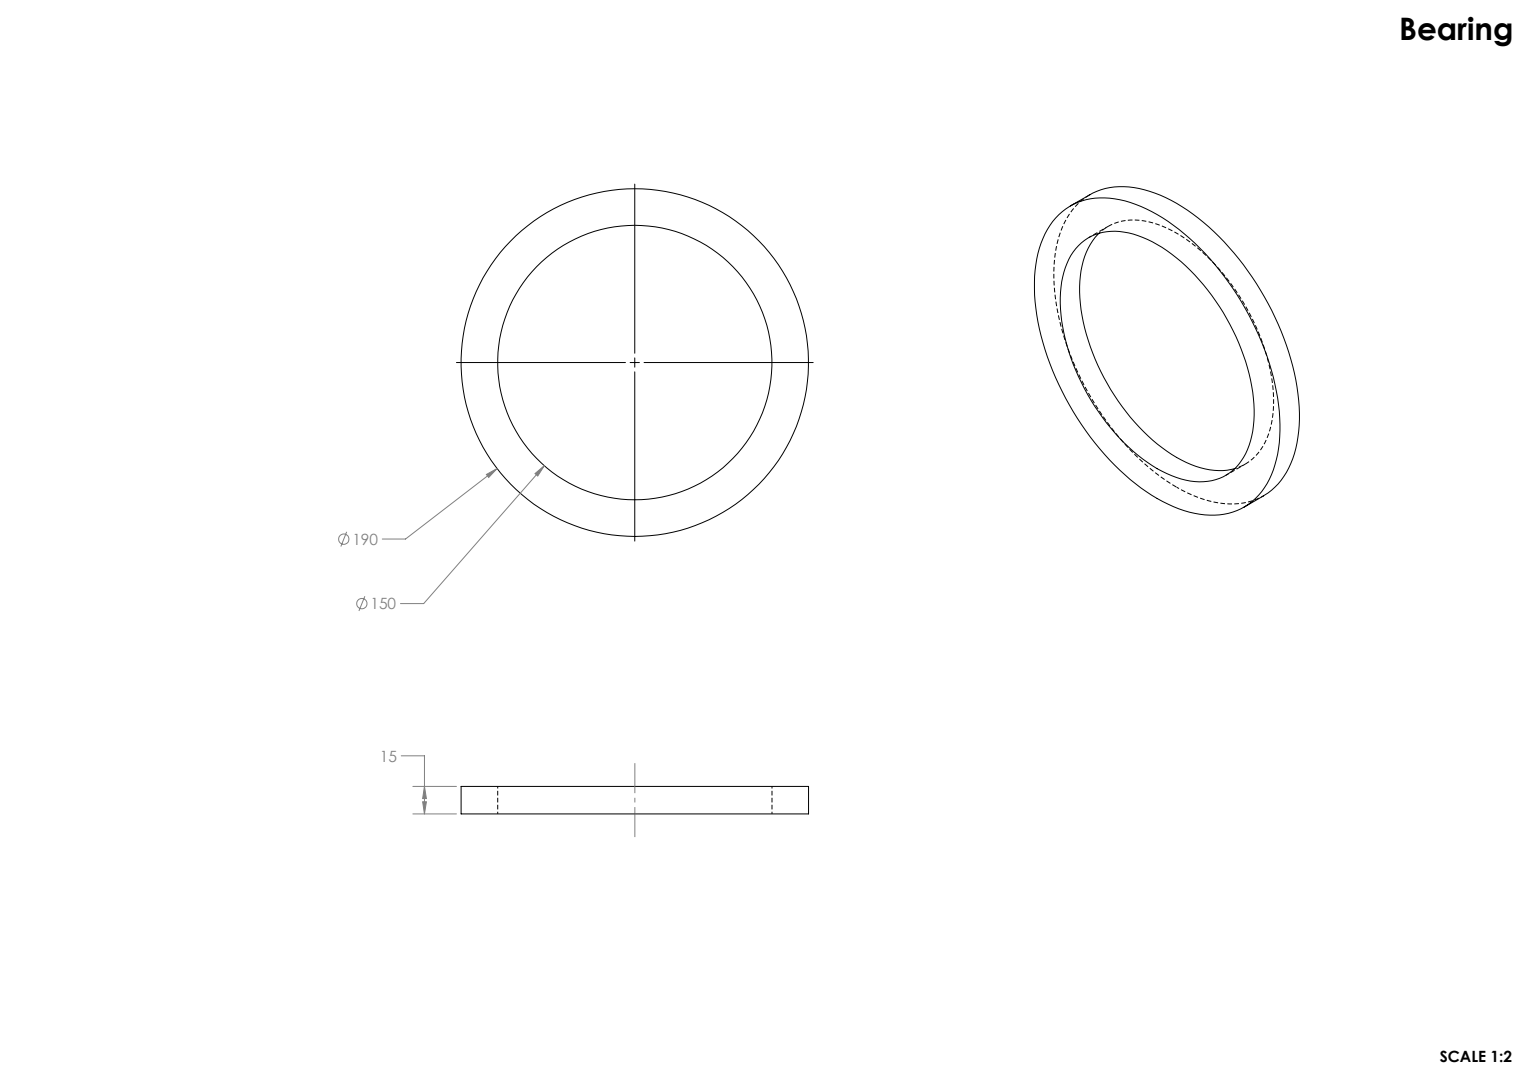
ISO-10303-21;
HEADER;
FILE_DESCRIPTION (('STEP AP214'),
    '1' );
FILE_NAME ('Bearing.step',
    '2026-10-28T15:55:38',
    ( '' ),
    ( '' ),
    'SwSTEP 2.0',
    'SolidWorks 2025',
    '' );
FILE_SCHEMA (( 'AUTOMOTIVE_DESIGN' ));
ENDSEC;

DATA;
#36=CYLINDRICAL_SURFACE ( 'NONE', #7648, 95.00000000000001421 ) ;
#43=DIRECTION ( 'NONE',  ( 0.000000000000000000, 0.000000000000000000, 1.000000000000000000 ) ) ;
#170=DIRECTION ( 'NONE',  ( 1.000000000000000000, 0.000000000000000000, 0.000000000000000000 ) ) ;
#319=CIRCLE ( 'NONE', #6386, 95.00000000000001421 ) ;
#459=DIRECTION ( 'NONE',  ( 1.000000000000000000, 0.000000000000000000, 0.000000000000000000 ) ) ;
#466=EDGE_LOOP ( 'NONE', ( #8090, #6345 ) ) ;
#470=EDGE_CURVE ( 'NONE', #8314, #877, #319, .T. ) ;
#507=AXIS2_PLACEMENT_3D ( 'NONE', #6558, #3976, #170 ) ;
#604=DIRECTION ( 'NONE',  ( -1.000000000000000000, 0.000000000000000000, 0.000000000000000000 ) ) ;
#729=CLOSED_SHELL ( 'NONE', ( #3816, #7770, #7786, #6914, #1126, #1756 ) ) ;
#772=AXIS2_PLACEMENT_3D ( 'NONE', #5605, #2410, #3654 ) ;
#778=ORIENTED_EDGE ( 'NONE', *, *, #5207, .F. ) ;
#813=PRODUCT_DEFINITION_SHAPE ( 'NONE', 'NONE',  #2910 ) ;
#833=ORIENTED_EDGE ( 'NONE', *, *, #6845, .F. ) ;
#877=VERTEX_POINT ( 'NONE', #3456 ) ;
#878=DIRECTION ( 'NONE',  ( 1.000000000000000000, 0.000000000000000000, -0.000000000000000000 ) ) ;
#883=ORIENTED_EDGE ( 'NONE', *, *, #2186, .T. ) ;
#931=MANIFOLD_SOLID_BREP ( 'Boss-Extrude1', #729 ) ;
#938=CIRCLE ( 'NONE', #2552, 75.00000000000001421 ) ;
#958=( NAMED_UNIT ( * ) PLANE_ANGLE_UNIT ( ) SI_UNIT ( $, .RADIAN. ) );
#968=AXIS2_PLACEMENT_3D ( 'NONE', #5784, #1269, #459 ) ;
#994=ORIENTED_EDGE ( 'NONE', *, *, #2184, .F. ) ;
#1126=ADVANCED_FACE ( 'NONE', ( #2059 ), #36, .T. ) ;
#1133=LINE ( 'NONE', #1260, #1871 ) ;
#1160=CYLINDRICAL_SURFACE ( 'NONE', #1942, 75.00000000000001421 ) ;
#1260=CARTESIAN_POINT ( 'NONE',  ( -75.00000000000001421, 0.000000000000000000, 15.00000000000000000 ) ) ;
#1269=DIRECTION ( 'NONE',  ( 0.000000000000000000, 0.000000000000000000, 1.000000000000000000 ) ) ;
#1270=CARTESIAN_POINT ( 'NONE',  ( -75.00000000000001421, 0.000000000000000000, 0.000000000000000000 ) ) ;
#1299=AXIS2_PLACEMENT_3D ( 'NONE', #5884, #1507, #5927 ) ;
#1321=FACE_OUTER_BOUND ( 'NONE', #2841, .T. ) ;
#1388=CARTESIAN_POINT ( 'NONE',  ( 0.000000000000000000, 0.000000000000000000, 0.000000000000000000 ) ) ;
#1448=EDGE_CURVE ( 'NONE', #5626, #4012, #7736, .T. ) ;
#1507=DIRECTION ( 'NONE',  ( 0.000000000000000000, 0.000000000000000000, 1.000000000000000000 ) ) ;
#1508=( LENGTH_UNIT ( ) NAMED_UNIT ( * ) SI_UNIT ( .MILLI., .METRE. ) );
#1514=FACE_OUTER_BOUND ( 'NONE', #2180, .T. ) ;
#1549=DIRECTION ( 'NONE',  ( 0.000000000000000000, 0.000000000000000000, 1.000000000000000000 ) ) ;
#1576=ORIENTED_EDGE ( 'NONE', *, *, #470, .T. ) ;
#1718=CARTESIAN_POINT ( 'NONE',  ( -95.00000000000001421, 0.000000000000000000, 15.00000000000000000 ) ) ;
#1719=DIRECTION ( 'NONE',  ( -0.000000000000000000, -0.000000000000000000, -1.000000000000000000 ) ) ;
#1756=ADVANCED_FACE ( 'NONE', ( #1321 ), #1160, .F. ) ;
#1871=VECTOR ( 'NONE', #1719, 1000.000000000000000 ) ;
#1901=ORIENTED_EDGE ( 'NONE', *, *, #6845, .T. ) ;
#1931=PLANE ( 'NONE',  #7835 ) ;
#1942=AXIS2_PLACEMENT_3D ( 'NONE', #4989, #5072, #604 ) ;
#1999=LINE ( 'NONE', #4491, #3203 ) ;
#2059=FACE_OUTER_BOUND ( 'NONE', #4783, .T. ) ;
#2128=ORIENTED_EDGE ( 'NONE', *, *, #5048, .F. ) ;
#2180=EDGE_LOOP ( 'NONE', ( #2394, #6230 ) ) ;
#2184=EDGE_CURVE ( 'NONE', #5018, #7120, #6621, .T. ) ;
#2186=EDGE_CURVE ( 'NONE', #4012, #5626, #5543, .T. ) ;
#2227=ADVANCED_BREP_SHAPE_REPRESENTATION ( '', ( #931, #1299 ), #5023 ) ;
#2394=ORIENTED_EDGE ( 'NONE', *, *, #4348, .F. ) ;
#2410=DIRECTION ( 'NONE',  ( -0.000000000000000000, -0.000000000000000000, -1.000000000000000000 ) ) ;
#2508=DIRECTION ( 'NONE',  ( -0.000000000000000000, -0.000000000000000000, -1.000000000000000000 ) ) ;
#2552=AXIS2_PLACEMENT_3D ( 'NONE', #7127, #4450, #7042 ) ;
#2554=DIRECTION ( 'NONE',  ( -1.000000000000000000, 0.000000000000000000, 0.000000000000000000 ) ) ;
#2597=EDGE_CURVE ( 'NONE', #5626, #5018, #1133, .T. ) ;
#2762=PLANE ( 'NONE',  #6990 ) ;
#2841=EDGE_LOOP ( 'NONE', ( #3155, #883, #6890, #833 ) ) ;
#2877=CARTESIAN_POINT ( 'NONE',  ( 0.000000000000000000, 0.000000000000000000, 15.00000000000000000 ) ) ;
#2910=PRODUCT_DEFINITION ( 'UNKNOWN', '', #4750, #4112 ) ;
#2967=AXIS2_PLACEMENT_3D ( 'NONE', #4370, #3835, #6926 ) ;
#3010=CARTESIAN_POINT ( 'NONE',  ( 75.00000000000001421, 9.184850993605150311E-15, 0.000000000000000000 ) ) ;
#3045=EDGE_CURVE ( 'NONE', #4012, #7120, #1999, .T. ) ;
#3070=SHAPE_DEFINITION_REPRESENTATION ( #813, #8061 ) ;
#3119=DIRECTION ( 'NONE',  ( 1.000000000000000000, 0.000000000000000000, 0.000000000000000000 ) ) ;
#3155=ORIENTED_EDGE ( 'NONE', *, *, #3045, .F. ) ;
#3167=CARTESIAN_POINT ( 'NONE',  ( 0.000000000000000000, 0.000000000000000000, 15.00000000000000000 ) ) ;
#3203=VECTOR ( 'NONE', #4288, 1000.000000000000000 ) ;
#3250=VERTEX_POINT ( 'NONE', #1718 ) ;
#3275=LINE ( 'NONE', #6536, #3329 ) ;
#3283=ORIENTED_EDGE ( 'NONE', *, *, #2184, .T. ) ;
#3329=VECTOR ( 'NONE', #4636, 1000.000000000000000 ) ;
#3350=VERTEX_POINT ( 'NONE', #6818 ) ;
#3360=APPLICATION_CONTEXT ( 'automotive_design' ) ;
#3380=AXIS2_PLACEMENT_3D ( 'NONE', #2877, #1549, #6614 ) ;
#3432=EDGE_LOOP ( 'NONE', ( #2128, #7481, #1576, #778 ) ) ;
#3456=CARTESIAN_POINT ( 'NONE',  ( -95.00000000000001421, 0.000000000000000000, 0.000000000000000000 ) ) ;
#3499=( NAMED_UNIT ( * ) SI_UNIT ( $, .STERADIAN. ) SOLID_ANGLE_UNIT ( ) );
#3584=CIRCLE ( 'NONE', #507, 95.00000000000001421 ) ;
#3654=DIRECTION ( 'NONE',  ( -1.000000000000000000, 0.000000000000000000, 0.000000000000000000 ) ) ;
#3709=ORIENTED_EDGE ( 'NONE', *, *, #5048, .T. ) ;
#3774=FACE_OUTER_BOUND ( 'NONE', #3432, .T. ) ;
#3816=ADVANCED_FACE ( 'NONE', ( #4362 ), #4965, .F. ) ;
#3835=DIRECTION ( 'NONE',  ( 0.000000000000000000, 0.000000000000000000, 1.000000000000000000 ) ) ;
#3976=DIRECTION ( 'NONE',  ( 0.000000000000000000, 0.000000000000000000, 1.000000000000000000 ) ) ;
#4012=VERTEX_POINT ( 'NONE', #5035 ) ;
#4090=MECHANICAL_DESIGN_GEOMETRIC_PRESENTATION_REPRESENTATION('',(#5733),#8020);
#4112=PRODUCT_DEFINITION_CONTEXT ( 'detailed design', #7435, 'design' ) ;
#4134=LINE ( 'NONE', #5418, #5387 ) ;
#4288=DIRECTION ( 'NONE',  ( -0.000000000000000000, -0.000000000000000000, -1.000000000000000000 ) ) ;
#4348=EDGE_CURVE ( 'NONE', #877, #8314, #3584, .T. ) ;
#4362=FACE_OUTER_BOUND ( 'NONE', #4998, .T. ) ;
#4370=CARTESIAN_POINT ( 'NONE',  ( 0.000000000000000000, 0.000000000000000000, 15.00000000000000000 ) ) ;
#4374=CARTESIAN_POINT ( 'NONE',  ( 0.000000000000000000, 0.000000000000000000, 15.00000000000000000 ) ) ;
#4429=CYLINDRICAL_SURFACE ( 'NONE', #5257, 95.00000000000001421 ) ;
#4439=DIRECTION ( 'NONE',  ( 0.000000000000000000, 0.000000000000000000, 1.000000000000000000 ) ) ;
#4450=DIRECTION ( 'NONE',  ( 0.000000000000000000, 0.000000000000000000, 1.000000000000000000 ) ) ;
#4491=CARTESIAN_POINT ( 'NONE',  ( 75.00000000000001421, 9.184850993605150311E-15, 15.00000000000000000 ) ) ;
#4503=CARTESIAN_POINT ( 'NONE',  ( 0.000000000000000000, 0.000000000000000000, 15.00000000000000000 ) ) ;
#4636=DIRECTION ( 'NONE',  ( -0.000000000000000000, -0.000000000000000000, -1.000000000000000000 ) ) ;
#4647=DIRECTION ( 'NONE',  ( 1.000000000000000000, 0.000000000000000000, -0.000000000000000000 ) ) ;
#4750=PRODUCT_DEFINITION_FORMATION_WITH_SPECIFIED_SOURCE ( 'ANY', '', #6807, .NOT_KNOWN. ) ;
#4783=EDGE_LOOP ( 'NONE', ( #7649, #6161, #7566, #5649 ) ) ;
#4810=EDGE_LOOP ( 'NONE', ( #3283, #1901 ) ) ;
#4821=( NAMED_UNIT ( * ) PLANE_ANGLE_UNIT ( ) SI_UNIT ( $, .RADIAN. ) );
#4921=PRODUCT_CONTEXT ( 'NONE', #3360, 'mechanical' ) ;
#4965=CYLINDRICAL_SURFACE ( 'NONE', #772, 75.00000000000001421 ) ;
#4989=CARTESIAN_POINT ( 'NONE',  ( 0.000000000000000000, 0.000000000000000000, 15.00000000000000000 ) ) ;
#4998=EDGE_LOOP ( 'NONE', ( #5801, #6492, #994, #6907 ) ) ;
#5018=VERTEX_POINT ( 'NONE', #1270 ) ;
#5023=( GEOMETRIC_REPRESENTATION_CONTEXT ( 3 ) GLOBAL_UNCERTAINTY_ASSIGNED_CONTEXT ( ( #6995 ) ) GLOBAL_UNIT_ASSIGNED_CONTEXT ( ( #5461, #958, #3499 ) ) REPRESENTATION_CONTEXT ( 'NONE', 'WORKASPACE' ) );
#5035=CARTESIAN_POINT ( 'NONE',  ( 75.00000000000001421, 9.184850993605150311E-15, 15.00000000000000000 ) ) ;
#5048=EDGE_CURVE ( 'NONE', #3350, #3250, #5095, .T. ) ;
#5072=DIRECTION ( 'NONE',  ( -0.000000000000000000, -0.000000000000000000, -1.000000000000000000 ) ) ;
#5095=CIRCLE ( 'NONE', #5369, 95.00000000000001421 ) ;
#5117=FACE_OUTER_BOUND ( 'NONE', #7436, .T. ) ;
#5207=EDGE_CURVE ( 'NONE', #3250, #877, #3275, .T. ) ;
#5257=AXIS2_PLACEMENT_3D ( 'NONE', #3167, #5754, #2554 ) ;
#5369=AXIS2_PLACEMENT_3D ( 'NONE', #4374, #7699, #3119 ) ;
#5387=VECTOR ( 'NONE', #7995, 1000.000000000000000 ) ;
#5408=DIRECTION ( 'NONE',  ( 1.000000000000000000, 0.000000000000000000, 0.000000000000000000 ) ) ;
#5418=CARTESIAN_POINT ( 'NONE',  ( 95.00000000000001421, 1.163414459189985801E-14, 15.00000000000000000 ) ) ;
#5461=( LENGTH_UNIT ( ) NAMED_UNIT ( * ) SI_UNIT ( .MILLI., .METRE. ) );
#5543=CIRCLE ( 'NONE', #2967, 75.00000000000001421 ) ;
#5589=CARTESIAN_POINT ( 'NONE',  ( 0.000000000000000000, 0.000000000000000000, 15.00000000000000000 ) ) ;
#5605=CARTESIAN_POINT ( 'NONE',  ( 0.000000000000000000, 0.000000000000000000, 15.00000000000000000 ) ) ;
#5626=VERTEX_POINT ( 'NONE', #7853 ) ;
#5649=ORIENTED_EDGE ( 'NONE', *, *, #4348, .T. ) ;
#5721=CARTESIAN_POINT ( 'NONE',  ( 0.000000000000000000, 0.000000000000000000, 15.00000000000000000 ) ) ;
#5733=STYLED_ITEM('',(#8400),#931);
#5754=DIRECTION ( 'NONE',  ( -0.000000000000000000, -0.000000000000000000, -1.000000000000000000 ) ) ;
#5784=CARTESIAN_POINT ( 'NONE',  ( 0.000000000000000000, 0.000000000000000000, 0.000000000000000000 ) ) ;
#5801=ORIENTED_EDGE ( 'NONE', *, *, #1448, .T. ) ;
#5884=CARTESIAN_POINT ( 'NONE',  ( 0.000000000000000000, 0.000000000000000000, 0.000000000000000000 ) ) ;
#5927=DIRECTION ( 'NONE',  ( 1.000000000000000000, 0.000000000000000000, 0.000000000000000000 ) ) ;
#5977=FACE_BOUND ( 'NONE', #4810, .T. ) ;
#6008=DIRECTION ( 'NONE',  ( 0.000000000000000000, 0.000000000000000000, 1.000000000000000000 ) ) ;
#6121=( NAMED_UNIT ( * ) SI_UNIT ( $, .STERADIAN. ) SOLID_ANGLE_UNIT ( ) );
#6161=ORIENTED_EDGE ( 'NONE', *, *, #7263, .F. ) ;
#6230=ORIENTED_EDGE ( 'NONE', *, *, #470, .F. ) ;
#6345=ORIENTED_EDGE ( 'NONE', *, *, #2186, .F. ) ;
#6377=CARTESIAN_POINT ( 'NONE',  ( 0.000000000000000000, 0.000000000000000000, 0.000000000000000000 ) ) ;
#6386=AXIS2_PLACEMENT_3D ( 'NONE', #6377, #7352, #5408 ) ;
#6394=UNCERTAINTY_MEASURE_WITH_UNIT (LENGTH_MEASURE( 1.000000000000000082E-05 ), #1508, 'distance_accuracy_value', 'NONE');
#6492=ORIENTED_EDGE ( 'NONE', *, *, #3045, .T. ) ;
#6536=CARTESIAN_POINT ( 'NONE',  ( -95.00000000000001421, 0.000000000000000000, 15.00000000000000000 ) ) ;
#6558=CARTESIAN_POINT ( 'NONE',  ( 0.000000000000000000, 0.000000000000000000, 0.000000000000000000 ) ) ;
#6614=DIRECTION ( 'NONE',  ( 1.000000000000000000, 0.000000000000000000, 0.000000000000000000 ) ) ;
#6621=CIRCLE ( 'NONE', #968, 75.00000000000001421 ) ;
#6723=CIRCLE ( 'NONE', #7825, 95.00000000000001421 ) ;
#6807=PRODUCT ( 'Bearing', 'Bearing', '', ( #4921 ) ) ;
#6818=CARTESIAN_POINT ( 'NONE',  ( 95.00000000000001421, 1.163414459189985801E-14, 15.00000000000000000 ) ) ;
#6845=EDGE_CURVE ( 'NONE', #7120, #5018, #938, .T. ) ;
#6890=ORIENTED_EDGE ( 'NONE', *, *, #2597, .T. ) ;
#6900=ORIENTED_EDGE ( 'NONE', *, *, #7263, .T. ) ;
#6907=ORIENTED_EDGE ( 'NONE', *, *, #2597, .F. ) ;
#6914=ADVANCED_FACE ( 'NONE', ( #1514, #5977 ), #2762, .F. ) ;
#6926=DIRECTION ( 'NONE',  ( 1.000000000000000000, 0.000000000000000000, 0.000000000000000000 ) ) ;
#6990=AXIS2_PLACEMENT_3D ( 'NONE', #1388, #6008, #878 ) ;
#6995=UNCERTAINTY_MEASURE_WITH_UNIT (LENGTH_MEASURE( 1.000000000000000082E-05 ), #5461, 'distance_accuracy_value', 'NONE');
#7018=DIRECTION ( 'NONE',  ( -1.000000000000000000, 0.000000000000000000, 0.000000000000000000 ) ) ;
#7042=DIRECTION ( 'NONE',  ( 1.000000000000000000, 0.000000000000000000, 0.000000000000000000 ) ) ;
#7120=VERTEX_POINT ( 'NONE', #3010 ) ;
#7127=CARTESIAN_POINT ( 'NONE',  ( 0.000000000000000000, 0.000000000000000000, 0.000000000000000000 ) ) ;
#7263=EDGE_CURVE ( 'NONE', #3250, #3350, #6723, .T. ) ;
#7352=DIRECTION ( 'NONE',  ( 0.000000000000000000, 0.000000000000000000, 1.000000000000000000 ) ) ;
#7435=APPLICATION_CONTEXT ( 'automotive_design' ) ;
#7436=EDGE_LOOP ( 'NONE', ( #6900, #3709 ) ) ;
#7481=ORIENTED_EDGE ( 'NONE', *, *, #7484, .T. ) ;
#7484=EDGE_CURVE ( 'NONE', #3350, #8314, #4134, .T. ) ;
#7566=ORIENTED_EDGE ( 'NONE', *, *, #5207, .T. ) ;
#7648=AXIS2_PLACEMENT_3D ( 'NONE', #4503, #2508, #7018 ) ;
#7649=ORIENTED_EDGE ( 'NONE', *, *, #7484, .F. ) ;
#7699=DIRECTION ( 'NONE',  ( 0.000000000000000000, 0.000000000000000000, 1.000000000000000000 ) ) ;
#7714=FACE_BOUND ( 'NONE', #466, .T. ) ;
#7736=CIRCLE ( 'NONE', #3380, 75.00000000000001421 ) ;
#7770=ADVANCED_FACE ( 'NONE', ( #3774 ), #4429, .T. ) ;
#7786=ADVANCED_FACE ( 'NONE', ( #5117, #7714 ), #1931, .T. ) ;
#7825=AXIS2_PLACEMENT_3D ( 'NONE', #5721, #4439, #8303 ) ;
#7835=AXIS2_PLACEMENT_3D ( 'NONE', #5589, #43, #4647 ) ;
#7853=CARTESIAN_POINT ( 'NONE',  ( -75.00000000000001421, 0.000000000000000000, 15.00000000000000000 ) ) ;
#7995=DIRECTION ( 'NONE',  ( -0.000000000000000000, -0.000000000000000000, -1.000000000000000000 ) ) ;
#8020=( GEOMETRIC_REPRESENTATION_CONTEXT ( 3 ) GLOBAL_UNCERTAINTY_ASSIGNED_CONTEXT ( ( #6394 ) ) GLOBAL_UNIT_ASSIGNED_CONTEXT ( ( #1508, #4821, #6121 ) ) REPRESENTATION_CONTEXT ( 'NONE', 'WORKASPACE' ) );
#8061=SHAPE_REPRESENTATION ( 'Bearing', ( #1299 ), #5023 ) ;
#8090=ORIENTED_EDGE ( 'NONE', *, *, #1448, .F. ) ;
#8215=SHAPE_REPRESENTATION_RELATIONSHIP ( 'NONE' , 'NONE' ,  #8061, #2227 ) ;
#8303=DIRECTION ( 'NONE',  ( 1.000000000000000000, 0.000000000000000000, 0.000000000000000000 ) ) ;
#8305=CARTESIAN_POINT ( 'NONE',  ( 95.00000000000001421, 1.163414459189985801E-14, 0.000000000000000000 ) ) ;
#8314=VERTEX_POINT ( 'NONE', #8305 ) ;
#8394=COLOUR_RGB('Grey',0.48,0.52,0.57);
#8395=FILL_AREA_STYLE_COLOUR('',#8394);
#8396=FILL_AREA_STYLE('',(#8395));
#8397=SURFACE_STYLE_FILL_AREA(#8396);
#8398=SURFACE_SIDE_STYLE('',(#8397));
#8399=SURFACE_STYLE_USAGE(.BOTH.,#8398);
#8400=PRESENTATION_STYLE_ASSIGNMENT((#8399));
ENDSEC;
END-ISO-10303-21;
